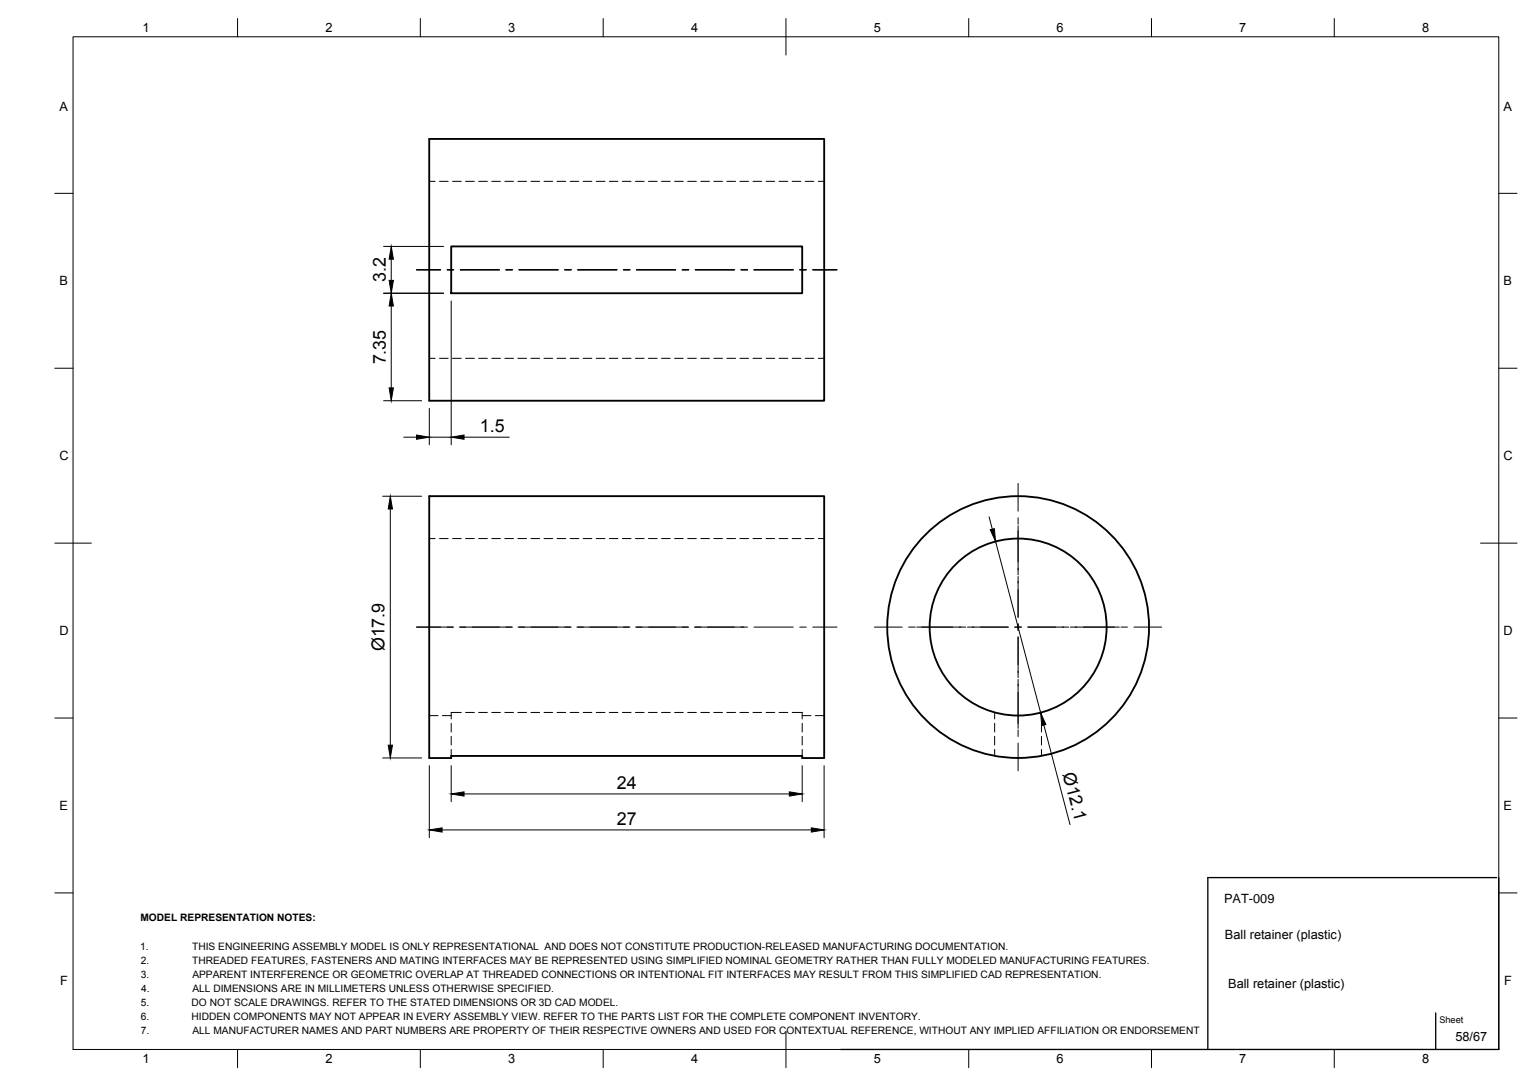
ISO-10303-21;
HEADER;
/* Generated by software containing ST-Developer
 * from STEP Tools, Inc. (www.steptools.com) 
 */

FILE_DESCRIPTION(
/* description */ ('Bell-crank linkage with push rods'),
/* implementation_level */ '2;1');

FILE_NAME(
/* name */ 'Ball retainer (plastic).step',
/* time_stamp */ '2026-10-28T03:25:15-07:00',
/* author */ (''),
/* organization */ (''),
/* preprocessor_version */ 'ST-DEVELOPER v20.2',
/* originating_system */ 'Autodesk Translation Framework v15.17.0.0',
/* authorisation */ '');

FILE_SCHEMA (('AUTOMOTIVE_DESIGN { 1 0 10303 214 3 1 1 }'));
ENDSEC;

DATA;
#10=MECHANICAL_DESIGN_GEOMETRIC_PRESENTATION_REPRESENTATION('',(#664),#16678);
#548=SHAPE_REPRESENTATION_RELATIONSHIP('SRR','None',#16971,#602);
#602=ADVANCED_BREP_SHAPE_REPRESENTATION('',(#724),#16676);
#664=STYLED_ITEM('',(#17284),#724);
#724=MANIFOLD_SOLID_BREP('Body1',#8856);
#961=FACE_BOUND('',#2508,.T.);
#962=FACE_BOUND('',#2510,.T.);
#963=FACE_BOUND('',#2512,.T.);
#964=FACE_BOUND('',#2514,.T.);
#1230=PLANE('',#10500);
#1231=PLANE('',#10503);
#1232=PLANE('',#10504);
#1233=PLANE('',#10507);
#1234=PLANE('',#10508);
#1235=PLANE('',#10513);
#1745=FACE_OUTER_BOUND('',#2503,.T.);
#1746=FACE_OUTER_BOUND('',#2504,.T.);
#1747=FACE_OUTER_BOUND('',#2505,.T.);
#1748=FACE_OUTER_BOUND('',#2506,.T.);
#1749=FACE_OUTER_BOUND('',#2507,.T.);
#1750=FACE_OUTER_BOUND('',#2509,.T.);
#1751=FACE_OUTER_BOUND('',#2511,.T.);
#1752=FACE_OUTER_BOUND('',#2513,.T.);
#2503=EDGE_LOOP('',(#7971,#7972,#7973,#7974));
#2504=EDGE_LOOP('',(#7975,#7976,#7977,#7978));
#2505=EDGE_LOOP('',(#7979,#7980,#7981,#7982));
#2506=EDGE_LOOP('',(#7983,#7984,#7985,#7986));
#2507=EDGE_LOOP('',(#7987));
#2508=EDGE_LOOP('',(#7988));
#2509=EDGE_LOOP('',(#7989,#7990,#7991,#7992));
#2510=EDGE_LOOP('',(#7993,#7994,#7995,#7996));
#2511=EDGE_LOOP('',(#7997));
#2512=EDGE_LOOP('',(#7998));
#2513=EDGE_LOOP('',(#7999,#8000,#8001,#8002));
#2514=EDGE_LOOP('',(#8003,#8004,#8005,#8006));
#3048=LINE('',#16362,#3597);
#3049=LINE('',#16365,#3598);
#3050=LINE('',#16368,#3599);
#3051=LINE('',#16370,#3600);
#3052=LINE('',#16371,#3601);
#3053=LINE('',#16377,#3602);
#3054=LINE('',#16379,#3603);
#3055=LINE('',#16380,#3604);
#3056=LINE('',#16389,#3605);
#3057=LINE('',#16394,#3606);
#3597=VECTOR('',#13242,1.);
#3598=VECTOR('',#13245,1.);
#3599=VECTOR('',#13248,1.);
#3600=VECTOR('',#13249,1.);
#3601=VECTOR('',#13250,1.);
#3602=VECTOR('',#13257,1.);
#3603=VECTOR('',#13260,1.);
#3604=VECTOR('',#13261,1.);
#3605=VECTOR('',#13272,0.895);
#3606=VECTOR('',#13279,0.605);
#4105=CIRCLE('',#10501,0.895);
#4106=CIRCLE('',#10502,0.605);
#4107=CIRCLE('',#10505,0.895);
#4108=CIRCLE('',#10506,0.605);
#4109=CIRCLE('',#10509,0.895);
#4110=CIRCLE('',#10510,0.605);
#4111=CIRCLE('',#10512,0.895);
#4112=CIRCLE('',#10514,0.605);
#4802=VERTEX_POINT('',#16358);
#4803=VERTEX_POINT('',#16359);
#4804=VERTEX_POINT('',#16361);
#4805=VERTEX_POINT('',#16363);
#4806=VERTEX_POINT('',#16367);
#4807=VERTEX_POINT('',#16369);
#4808=VERTEX_POINT('',#16373);
#4809=VERTEX_POINT('',#16375);
#4810=VERTEX_POINT('',#16382);
#4811=VERTEX_POINT('',#16384);
#4812=VERTEX_POINT('',#16387);
#4813=VERTEX_POINT('',#16391);
#5863=EDGE_CURVE('',#4802,#4803,#4105,.T.);
#5864=EDGE_CURVE('',#4804,#4802,#3048,.T.);
#5865=EDGE_CURVE('',#4805,#4804,#4106,.T.);
#5866=EDGE_CURVE('',#4803,#4805,#3049,.T.);
#5867=EDGE_CURVE('',#4803,#4806,#3050,.T.);
#5868=EDGE_CURVE('',#4807,#4805,#3051,.T.);
#5869=EDGE_CURVE('',#4807,#4806,#3052,.T.);
#5870=EDGE_CURVE('',#4806,#4808,#4107,.T.);
#5871=EDGE_CURVE('',#4809,#4807,#4108,.T.);
#5872=EDGE_CURVE('',#4808,#4809,#3053,.T.);
#5873=EDGE_CURVE('',#4808,#4802,#3054,.T.);
#5874=EDGE_CURVE('',#4804,#4809,#3055,.T.);
#5875=EDGE_CURVE('',#4810,#4810,#4109,.T.);
#5876=EDGE_CURVE('',#4811,#4811,#4110,.T.);
#5877=EDGE_CURVE('',#4812,#4812,#4111,.T.);
#5878=EDGE_CURVE('',#4812,#4810,#3056,.T.);
#5879=EDGE_CURVE('',#4813,#4813,#4112,.T.);
#5880=EDGE_CURVE('',#4813,#4811,#3057,.T.);
#7971=ORIENTED_EDGE('',*,*,#5863,.F.);
#7972=ORIENTED_EDGE('',*,*,#5864,.F.);
#7973=ORIENTED_EDGE('',*,*,#5865,.F.);
#7974=ORIENTED_EDGE('',*,*,#5866,.F.);
#7975=ORIENTED_EDGE('',*,*,#5867,.F.);
#7976=ORIENTED_EDGE('',*,*,#5866,.T.);
#7977=ORIENTED_EDGE('',*,*,#5868,.F.);
#7978=ORIENTED_EDGE('',*,*,#5869,.T.);
#7979=ORIENTED_EDGE('',*,*,#5870,.F.);
#7980=ORIENTED_EDGE('',*,*,#5869,.F.);
#7981=ORIENTED_EDGE('',*,*,#5871,.F.);
#7982=ORIENTED_EDGE('',*,*,#5872,.F.);
#7983=ORIENTED_EDGE('',*,*,#5873,.F.);
#7984=ORIENTED_EDGE('',*,*,#5872,.T.);
#7985=ORIENTED_EDGE('',*,*,#5874,.F.);
#7986=ORIENTED_EDGE('',*,*,#5864,.T.);
#7987=ORIENTED_EDGE('',*,*,#5875,.F.);
#7988=ORIENTED_EDGE('',*,*,#5876,.T.);
#7989=ORIENTED_EDGE('',*,*,#5877,.F.);
#7990=ORIENTED_EDGE('',*,*,#5878,.T.);
#7991=ORIENTED_EDGE('',*,*,#5875,.T.);
#7992=ORIENTED_EDGE('',*,*,#5878,.F.);
#7993=ORIENTED_EDGE('',*,*,#5870,.T.);
#7994=ORIENTED_EDGE('',*,*,#5873,.T.);
#7995=ORIENTED_EDGE('',*,*,#5863,.T.);
#7996=ORIENTED_EDGE('',*,*,#5867,.T.);
#7997=ORIENTED_EDGE('',*,*,#5877,.T.);
#7998=ORIENTED_EDGE('',*,*,#5879,.F.);
#7999=ORIENTED_EDGE('',*,*,#5879,.T.);
#8000=ORIENTED_EDGE('',*,*,#5880,.T.);
#8001=ORIENTED_EDGE('',*,*,#5876,.F.);
#8002=ORIENTED_EDGE('',*,*,#5880,.F.);
#8003=ORIENTED_EDGE('',*,*,#5871,.T.);
#8004=ORIENTED_EDGE('',*,*,#5868,.T.);
#8005=ORIENTED_EDGE('',*,*,#5865,.T.);
#8006=ORIENTED_EDGE('',*,*,#5874,.T.);
#8268=CYLINDRICAL_SURFACE('',#10511,0.895);
#8269=CYLINDRICAL_SURFACE('',#10515,0.605);
#8770=ADVANCED_FACE('',(#1745),#1230,.F.);
#8771=ADVANCED_FACE('',(#1746),#1231,.F.);
#8772=ADVANCED_FACE('',(#1747),#1232,.F.);
#8773=ADVANCED_FACE('',(#1748),#1233,.F.);
#8774=ADVANCED_FACE('',(#1749,#961),#1234,.T.);
#8775=ADVANCED_FACE('',(#1750,#962),#8268,.T.);
#8776=ADVANCED_FACE('',(#1751,#963),#1235,.T.);
#8777=ADVANCED_FACE('',(#1752,#964),#8269,.F.);
#8856=CLOSED_SHELL('',(#8770,#8771,#8772,#8773,#8774,#8775,#8776,#8777));
#10499=AXIS2_PLACEMENT_3D('',#16356,#13236,#13237);
#10500=AXIS2_PLACEMENT_3D('',#16357,#13238,#13239);
#10501=AXIS2_PLACEMENT_3D('',#16360,#13240,#13241);
#10502=AXIS2_PLACEMENT_3D('',#16364,#13243,#13244);
#10503=AXIS2_PLACEMENT_3D('',#16366,#13246,#13247);
#10504=AXIS2_PLACEMENT_3D('',#16372,#13251,#13252);
#10505=AXIS2_PLACEMENT_3D('',#16374,#13253,#13254);
#10506=AXIS2_PLACEMENT_3D('',#16376,#13255,#13256);
#10507=AXIS2_PLACEMENT_3D('',#16378,#13258,#13259);
#10508=AXIS2_PLACEMENT_3D('',#16381,#13262,#13263);
#10509=AXIS2_PLACEMENT_3D('',#16383,#13264,#13265);
#10510=AXIS2_PLACEMENT_3D('',#16385,#13266,#13267);
#10511=AXIS2_PLACEMENT_3D('',#16386,#13268,#13269);
#10512=AXIS2_PLACEMENT_3D('',#16388,#13270,#13271);
#10513=AXIS2_PLACEMENT_3D('',#16390,#13273,#13274);
#10514=AXIS2_PLACEMENT_3D('',#16392,#13275,#13276);
#10515=AXIS2_PLACEMENT_3D('',#16393,#13277,#13278);
#13236=DIRECTION('axis',(0.,0.,1.));
#13237=DIRECTION('refdir',(1.,0.,0.));
#13238=DIRECTION('center_axis',(0.,1.,0.));
#13239=DIRECTION('ref_axis',(0.,0.,1.));
#13240=DIRECTION('center_axis',(0.,1.,0.));
#13241=DIRECTION('ref_axis',(1.,0.,0.));
#13242=DIRECTION('',(1.,0.,0.));
#13243=DIRECTION('center_axis',(0.,-1.,0.));
#13244=DIRECTION('ref_axis',(1.,0.,0.));
#13245=DIRECTION('',(-1.,0.,0.));
#13246=DIRECTION('center_axis',(0.,0.,-1.));
#13247=DIRECTION('ref_axis',(-1.,0.,0.));
#13248=DIRECTION('',(0.,-1.,0.));
#13249=DIRECTION('',(0.,1.,0.));
#13250=DIRECTION('',(1.,0.,0.));
#13251=DIRECTION('center_axis',(0.,-1.,0.));
#13252=DIRECTION('ref_axis',(0.,0.,-1.));
#13253=DIRECTION('center_axis',(0.,-1.,0.));
#13254=DIRECTION('ref_axis',(1.,0.,0.));
#13255=DIRECTION('center_axis',(0.,1.,0.));
#13256=DIRECTION('ref_axis',(1.,0.,0.));
#13257=DIRECTION('',(-1.,0.,0.));
#13258=DIRECTION('center_axis',(0.,0.,1.));
#13259=DIRECTION('ref_axis',(1.,0.,0.));
#13260=DIRECTION('',(0.,1.,0.));
#13261=DIRECTION('',(0.,-1.,0.));
#13262=DIRECTION('center_axis',(0.,1.,0.));
#13263=DIRECTION('ref_axis',(0.,0.,1.));
#13264=DIRECTION('center_axis',(0.,-1.,0.));
#13265=DIRECTION('ref_axis',(1.,0.,0.));
#13266=DIRECTION('center_axis',(0.,-1.,0.));
#13267=DIRECTION('ref_axis',(1.,0.,0.));
#13268=DIRECTION('center_axis',(0.,-1.,0.));
#13269=DIRECTION('ref_axis',(1.,0.,0.));
#13270=DIRECTION('center_axis',(0.,-1.,0.));
#13271=DIRECTION('ref_axis',(1.,0.,0.));
#13272=DIRECTION('',(0.,1.,0.));
#13273=DIRECTION('center_axis',(0.,-1.,0.));
#13274=DIRECTION('ref_axis',(0.,0.,-1.));
#13275=DIRECTION('center_axis',(0.,-1.,0.));
#13276=DIRECTION('ref_axis',(1.,0.,0.));
#13277=DIRECTION('center_axis',(0.,-1.,0.));
#13278=DIRECTION('ref_axis',(1.,0.,0.));
#13279=DIRECTION('',(0.,1.,0.));
#16356=CARTESIAN_POINT('',(0.,0.,0.));
#16357=CARTESIAN_POINT('Origin',(0.75,1.2,0.));
#16358=CARTESIAN_POINT('',(0.880582193778639,1.2,0.16));
#16359=CARTESIAN_POINT('',(0.880582193778639,1.2,-0.16));
#16360=CARTESIAN_POINT('Origin',(0.,1.2,0.));
#16361=CARTESIAN_POINT('',(0.583459510163302,1.2,0.16));
#16362=CARTESIAN_POINT('',(0.57,1.2,0.16));
#16363=CARTESIAN_POINT('',(0.583459510163302,1.2,-0.16));
#16364=CARTESIAN_POINT('Origin',(0.,1.2,0.));
#16365=CARTESIAN_POINT('',(0.93,1.2,-0.16));
#16366=CARTESIAN_POINT('Origin',(0.93,0.,-0.16));
#16367=CARTESIAN_POINT('',(0.880582193778639,-1.2,-0.16));
#16368=CARTESIAN_POINT('',(0.880582193778639,0.,-0.16));
#16369=CARTESIAN_POINT('',(0.583459510163302,-1.2,-0.16));
#16370=CARTESIAN_POINT('',(0.583459510163302,0.,-0.16));
#16371=CARTESIAN_POINT('',(0.93,-1.2,-0.16));
#16372=CARTESIAN_POINT('Origin',(0.75,-1.2,0.));
#16373=CARTESIAN_POINT('',(0.880582193778639,-1.2,0.16));
#16374=CARTESIAN_POINT('Origin',(0.,-1.2,0.));
#16375=CARTESIAN_POINT('',(0.583459510163302,-1.2,0.16));
#16376=CARTESIAN_POINT('Origin',(0.,-1.2,0.));
#16377=CARTESIAN_POINT('',(0.57,-1.2,0.16));
#16378=CARTESIAN_POINT('Origin',(0.57,0.,0.16));
#16379=CARTESIAN_POINT('',(0.880582193778639,0.,0.16));
#16380=CARTESIAN_POINT('',(0.583459510163302,0.,0.16));
#16381=CARTESIAN_POINT('Origin',(0.895,1.35,0.));
#16382=CARTESIAN_POINT('',(-0.895,1.35,-1.09605888523688E-16));
#16383=CARTESIAN_POINT('Origin',(0.,1.35,0.));
#16384=CARTESIAN_POINT('',(-0.605,1.35,-7.40911313484149E-17));
#16385=CARTESIAN_POINT('Origin',(0.,1.35,0.));
#16386=CARTESIAN_POINT('Origin',(0.,0.,0.));
#16387=CARTESIAN_POINT('',(-0.895,-1.35,-1.09605888523688E-16));
#16388=CARTESIAN_POINT('Origin',(0.,-1.35,0.));
#16389=CARTESIAN_POINT('',(-0.895,0.,-1.09605888523688E-16));
#16390=CARTESIAN_POINT('Origin',(0.605,-1.35,0.));
#16391=CARTESIAN_POINT('',(-0.605,-1.35,-7.40911313484149E-17));
#16392=CARTESIAN_POINT('Origin',(0.,-1.35,0.));
#16393=CARTESIAN_POINT('Origin',(0.,0.,0.));
#16394=CARTESIAN_POINT('',(-0.605,0.,-7.40911313484149E-17));
#16612=UNCERTAINTY_MEASURE_WITH_UNIT(LENGTH_MEASURE(0.001),#16679,
'DISTANCE_ACCURACY_VALUE',
'Maximum model space distance between geometric entities at asserted c
onnectivities');
#16614=UNCERTAINTY_MEASURE_WITH_UNIT(LENGTH_MEASURE(0.001),#16679,
'DISTANCE_ACCURACY_VALUE',
'Maximum model space distance between geometric entities at asserted c
onnectivities');
#16676=(
GEOMETRIC_REPRESENTATION_CONTEXT(3)
GLOBAL_UNCERTAINTY_ASSIGNED_CONTEXT((#16612))
GLOBAL_UNIT_ASSIGNED_CONTEXT((#16679,#16681,#16682))
REPRESENTATION_CONTEXT('','3D')
);
#16678=(
GEOMETRIC_REPRESENTATION_CONTEXT(3)
GLOBAL_UNCERTAINTY_ASSIGNED_CONTEXT((#16614))
GLOBAL_UNIT_ASSIGNED_CONTEXT((#16679,#16681,#16682))
REPRESENTATION_CONTEXT('','3D')
);
#16679=(
LENGTH_UNIT()
NAMED_UNIT(*)
SI_UNIT(.CENTI.,.METRE.)
);
#16681=(
NAMED_UNIT(*)
PLANE_ANGLE_UNIT()
SI_UNIT($,.RADIAN.)
);
#16682=(
NAMED_UNIT(*)
SI_UNIT($,.STERADIAN.)
SOLID_ANGLE_UNIT()
);
#16744=SHAPE_DEFINITION_REPRESENTATION(#16818,#16971);
#16818=PRODUCT_DEFINITION_SHAPE('',$,#17035);
#16971=SHAPE_REPRESENTATION('',(#10499),#16676);
#16973=PRODUCT_DEFINITION_CONTEXT('part definition',#17164,'design');
#17035=PRODUCT_DEFINITION('Ball retainer (plastic)',
'Ball retainer (plastic)',#17098,#16973);
#17098=PRODUCT_DEFINITION_FORMATION('',$,#17227);
#17164=APPLICATION_CONTEXT(
'Core Data for Automotive Mechanical Design Process');
#17165=PRODUCT_CONTEXT('part definition',#17164,'mechanical');
#17227=PRODUCT('Ball retainer (plastic)','Ball retainer (plastic)',
'Ball retainer (plastic)',(#17165));
#17278=COLOUR_RGB('Sky Blue',0.24,0.69,0.87);
#17279=FILL_AREA_STYLE_COLOUR('',#17278);
#17280=FILL_AREA_STYLE('',(#17279));
#17281=SURFACE_STYLE_FILL_AREA(#17280);
#17282=SURFACE_SIDE_STYLE('',(#17281));
#17283=SURFACE_STYLE_USAGE(.BOTH.,#17282);
#17284=PRESENTATION_STYLE_ASSIGNMENT((#17283));
ENDSEC;
END-ISO-10303-21;
